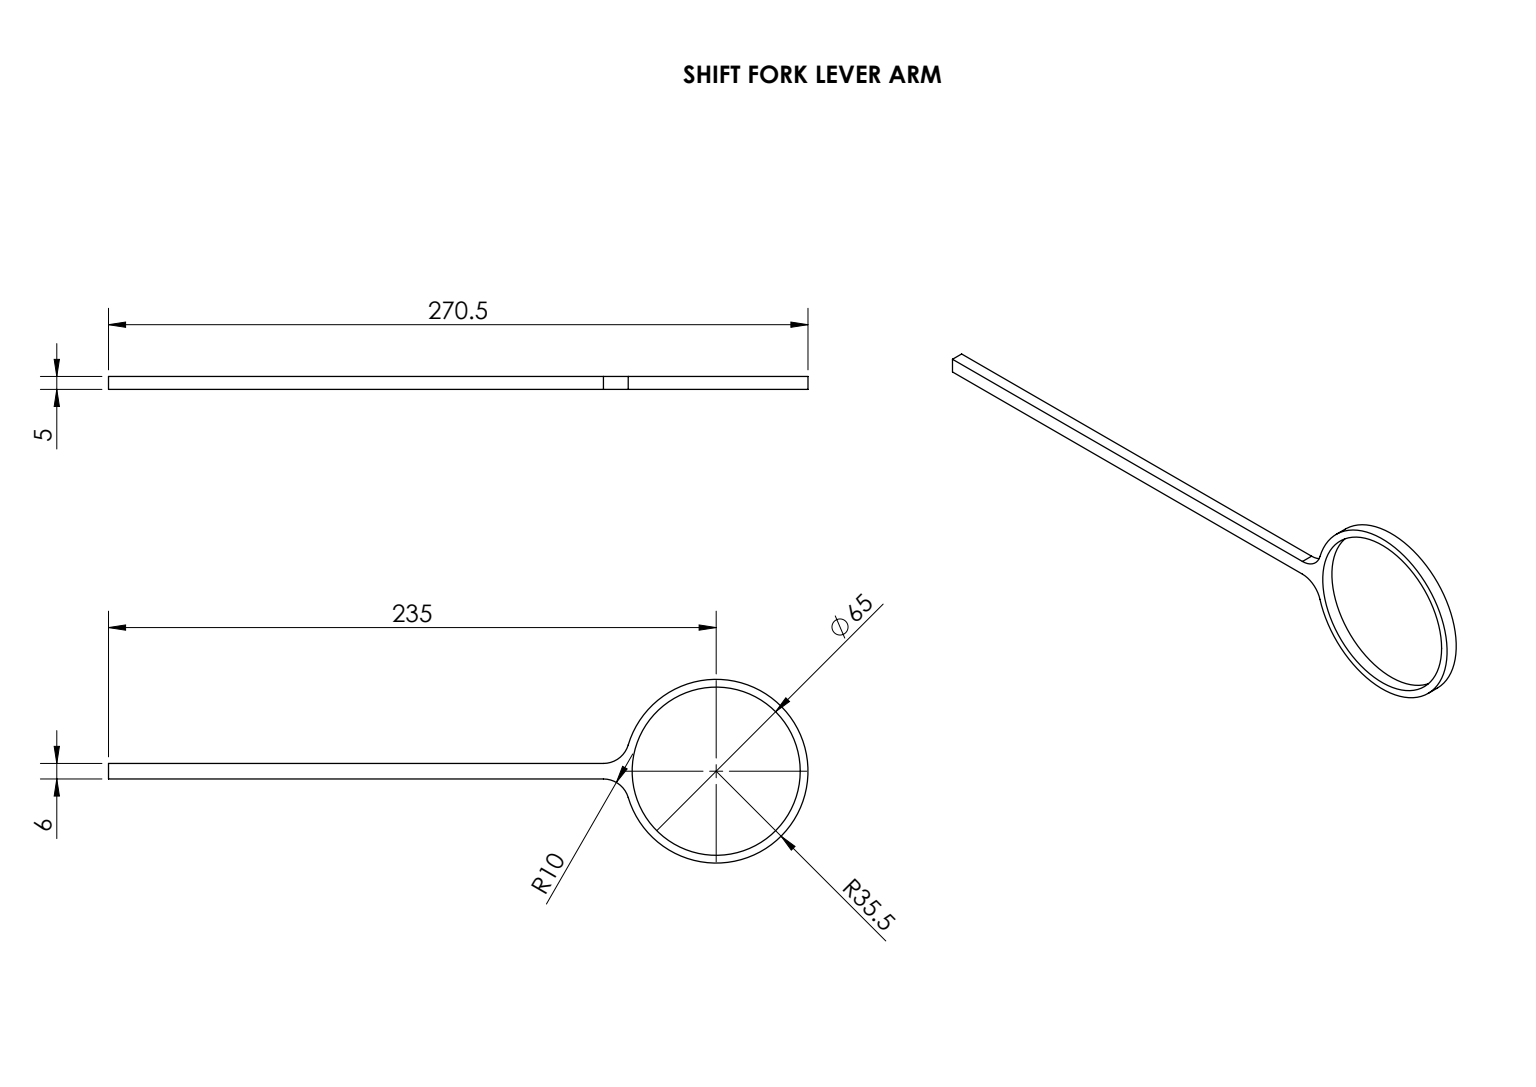
ISO-10303-21;
HEADER;
FILE_DESCRIPTION (('STEP AP214'),
    '1' );
FILE_NAME ('Shift Fork Lever Arm.step',
    '2026-10-08T09:53:37',
    ( '' ),
    ( '' ),
    'SwSTEP 2.0',
    'SolidWorks 2026',
    '' );
FILE_SCHEMA (( 'AUTOMOTIVE_DESIGN' ));
ENDSEC;

DATA;
#279=MECHANICAL_DESIGN_GEOMETRIC_PRESENTATION_REPRESENTATION('',(#31450),#13423);
#493=EDGE_CURVE ( 'NONE', #50397, #40961, #31739, .T. ) ;
#506=EDGE_LOOP ( 'NONE', ( #47657, #21524 ) ) ;
#1089=ORIENTED_EDGE ( 'NONE', *, *, #58225, .F. ) ;
#1094=VERTEX_POINT ( 'NONE', #69858 ) ;
#1250=ORIENTED_EDGE ( 'NONE', *, *, #69986, .F. ) ;
#1371=CARTESIAN_POINT ( 'NONE',  ( 0.000000000000000000, -120.0000000000000000, 2.500000000000000000 ) ) ;
#1832=ORIENTED_EDGE ( 'NONE', *, *, #65900, .T. ) ;
#1851=CARTESIAN_POINT ( 'NONE',  ( -35.37301231164799731, -123.0000000000000142, 2.500000000000000000 ) ) ;
#2124=PRESENTATION_STYLE_ASSIGNMENT (( #17159 ) ) ;
#2378=DIRECTION ( 'NONE',  ( 0.000000000000000000, 0.000000000000000000, -1.000000000000000000 ) ) ;
#2416=( NAMED_UNIT ( * ) PLANE_ANGLE_UNIT ( ) SI_UNIT ( $, .RADIAN. ) );
#2539=CARTESIAN_POINT ( 'NONE',  ( -43.60332556124591008, -133.0000000000000000, 2.500000000000002220 ) ) ;
#2571=DIRECTION ( 'NONE',  ( 0.000000000000000000, 0.000000000000000000, 1.000000000000000000 ) ) ;
#2729=ORIENTED_EDGE ( 'NONE', *, *, #17511, .F. ) ;
#2903=DIRECTION ( 'NONE',  ( -0.000000000000000000, -0.000000000000000000, -1.000000000000000000 ) ) ;
#2976=CARTESIAN_POINT ( 'NONE',  ( -43.60332556124591008, -123.0000000000000142, 2.500000000000000000 ) ) ;
#3170=PRODUCT_DEFINITION_SHAPE ( 'NONE', 'NONE',  #3585 ) ;
#3188=FACE_OUTER_BOUND ( 'NONE', #56711, .T. ) ;
#3275=ORIENTED_EDGE ( 'NONE', *, *, #38816, .F. ) ;
#3585=PRODUCT_DEFINITION ( 'UNKNOWN', '', #40042, #37882 ) ;
#3925=CARTESIAN_POINT ( 'NONE',  ( 0.000000000000000000, -120.0000000000000000, -2.500000000000000000 ) ) ;
#4365=EDGE_CURVE ( 'NONE', #9063, #35752, #34989, .T. ) ;
#4378=ORIENTED_EDGE ( 'NONE', *, *, #60273, .T. ) ;
#4546=VERTEX_POINT ( 'NONE', #31183 ) ;
#5317=ORIENTED_EDGE ( 'NONE', *, *, #5543, .T. ) ;
#5519=CIRCLE ( 'NONE', #39091, 35.50000000000000711 ) ;
#5524=FILL_AREA_STYLE ('',( #57018 ) ) ;
#5543=EDGE_CURVE ( 'NONE', #40961, #24049, #31285, .T. ) ;
#5914=AXIS2_PLACEMENT_3D ( 'NONE', #72472, #61583, #21719 ) ;
#6313=ORIENTED_EDGE ( 'NONE', *, *, #61943, .F. ) ;
#6345=CYLINDRICAL_SURFACE ( 'NONE', #60879, 10.00000000000000178 ) ;
#6694=CARTESIAN_POINT ( 'NONE',  ( 0.000000000000000000, -120.0000000000000000, 2.500000000000000000 ) ) ;
#6741=AXIS2_PLACEMENT_3D ( 'NONE', #9368, #48121, #71037 ) ;
#6882=DIRECTION ( 'NONE',  ( -0.000000000000000000, -0.000000000000000000, -1.000000000000000000 ) ) ;
#6961=AXIS2_PLACEMENT_3D ( 'NONE', #15987, #28005, #39680 ) ;
#7060=EDGE_CURVE ( 'NONE', #1094, #43028, #54701, .T. ) ;
#7091=DIRECTION ( 'NONE',  ( -0.000000000000000000, -0.000000000000000000, -1.000000000000000000 ) ) ;
#7468=EDGE_CURVE ( 'NONE', #56318, #9063, #47331, .T. ) ;
#7900=DIRECTION ( 'NONE',  ( -0.000000000000000000, -0.000000000000000000, -1.000000000000000000 ) ) ;
#7939=ORIENTED_EDGE ( 'NONE', *, *, #55262, .F. ) ;
#7967=CARTESIAN_POINT ( 'NONE',  ( -235.0000123116479926, -123.0000000000000284, 2.500000000000000000 ) ) ;
#8007=SHAPE_REPRESENTATION_RELATIONSHIP ( 'NONE' , 'NONE' ,  #54059, #64162 ) ;
#8296=AXIS2_PLACEMENT_3D ( 'NONE', #54037, #2571, #25454 ) ;
#8331=ORIENTED_EDGE ( 'NONE', *, *, #55262, .T. ) ;
#8584=ORIENTED_EDGE ( 'NONE', *, *, #493, .F. ) ;
#8605=ORIENTED_EDGE ( 'NONE', *, *, #53404, .F. ) ;
#8753=( NAMED_UNIT ( * ) SI_UNIT ( $, .STERADIAN. ) SOLID_ANGLE_UNIT ( ) );
#9036=DIRECTION ( 'NONE',  ( -1.000000000000000000, -1.390371824233641368E-16, 0.000000000000000000 ) ) ;
#9063=VERTEX_POINT ( 'NONE', #38613 ) ;
#9368=CARTESIAN_POINT ( 'NONE',  ( 0.000000000000000000, -89.50000000000000000, 2.500000000000000000 ) ) ;
#9389=AXIS2_PLACEMENT_3D ( 'NONE', #63819, #22857, #29567 ) ;
#9403=CARTESIAN_POINT ( 'NONE',  ( -35.37301231164799731, -117.0000000000000000, 2.500000000000000000 ) ) ;
#9425=AXIS2_PLACEMENT_3D ( 'NONE', #65440, #18807, #41748 ) ;
#9496=AXIS2_PLACEMENT_3D ( 'NONE', #7967, #30884, #2378 ) ;
#9669=CARTESIAN_POINT ( 'NONE',  ( -43.60332556124591719, -107.0000000000000000, -2.500000000000002220 ) ) ;
#10522=STYLED_ITEM ( 'NONE', ( #2124 ), #12416 ) ;
#11005=PRODUCT ( 'Shift Fork Lever Arm', 'Shift Fork Lever Arm', '', ( #62921 ) ) ;
#11567=DIRECTION ( 'NONE',  ( 1.000000000000000000, 0.000000000000000000, 0.000000000000000000 ) ) ;
#11920=FACE_OUTER_BOUND ( 'NONE', #33954, .T. ) ;
#12163=( NAMED_UNIT ( * ) PLANE_ANGLE_UNIT ( ) SI_UNIT ( $, .RADIAN. ) );
#12416=MANIFOLD_SOLID_BREP ( 'Fillet1', #39184 ) ;
#12418=DIRECTION ( 'NONE',  ( -0.000000000000000000, -0.000000000000000000, -1.000000000000000000 ) ) ;
#12755=CARTESIAN_POINT ( 'NONE',  ( -34.02017708624681092, -109.8571428571428470, -2.500000000000000000 ) ) ;
#12885=VECTOR ( 'NONE', #6882, 1000.000000000000000 ) ;
#12983=DIRECTION ( 'NONE',  ( 0.000000000000000000, 0.000000000000000000, -1.000000000000000000 ) ) ;
#13364=CARTESIAN_POINT ( 'NONE',  ( -43.60332556124591719, -107.0000000000000000, 2.500000000000002220 ) ) ;
#13423=( GEOMETRIC_REPRESENTATION_CONTEXT ( 3 ) GLOBAL_UNCERTAINTY_ASSIGNED_CONTEXT ( ( #50455 ) ) GLOBAL_UNIT_ASSIGNED_CONTEXT ( ( #48956, #2416, #59522 ) ) REPRESENTATION_CONTEXT ( 'NONE', 'WORKASPACE' ) );
#13429=FACE_OUTER_BOUND ( 'NONE', #53169, .T. ) ;
#13605=PLANE ( 'NONE',  #9496 ) ;
#13638=PRESENTATION_STYLE_ASSIGNMENT (( #53869 ) ) ;
#13734=CARTESIAN_POINT ( 'NONE',  ( 32.50000000000000000, -120.0000000000000000, -2.500000000000000000 ) ) ;
#13827=FACE_OUTER_BOUND ( 'NONE', #32175, .T. ) ;
#14831=ORIENTED_EDGE ( 'NONE', *, *, #7468, .F. ) ;
#15138=CARTESIAN_POINT ( 'NONE',  ( -235.0000123116479926, -117.0000000000000142, -2.500000000000000000 ) ) ;
#15313=ORIENTED_EDGE ( 'NONE', *, *, #60273, .F. ) ;
#15737=DIRECTION ( 'NONE',  ( 0.000000000000000000, 0.000000000000000000, 1.000000000000000000 ) ) ;
#15987=CARTESIAN_POINT ( 'NONE',  ( 0.000000000000000000, -120.0000000000000000, -2.500000000000000000 ) ) ;
#16227=CARTESIAN_POINT ( 'NONE',  ( -43.60332556124591008, -133.0000000000000000, -2.500000000000002220 ) ) ;
#16229=VECTOR ( 'NONE', #7091, 1000.000000000000000 ) ;
#16483=ORIENTED_EDGE ( 'NONE', *, *, #53404, .T. ) ;
#16593=VECTOR ( 'NONE', #2903, 1000.000000000000000 ) ;
#17053=DIRECTION ( 'NONE',  ( 0.000000000000000000, 0.000000000000000000, 1.000000000000000000 ) ) ;
#17123=ORIENTED_EDGE ( 'NONE', *, *, #45687, .T. ) ;
#17159=SURFACE_STYLE_USAGE ( .BOTH. , #45751 ) ;
#17215=ORIENTED_EDGE ( 'NONE', *, *, #73567, .F. ) ;
#17511=EDGE_CURVE ( 'NONE', #56318, #50947, #63362, .T. ) ;
#17619=DIRECTION ( 'NONE',  ( 1.000000000000000000, 0.000000000000000000, 0.000000000000000000 ) ) ;
#17699=CIRCLE ( 'NONE', #29699, 10.00000000000000178 ) ;
#18203=VECTOR ( 'NONE', #7900, 1000.000000000000000 ) ;
#18807=DIRECTION ( 'NONE',  ( -0.000000000000000000, -0.000000000000000000, -1.000000000000000000 ) ) ;
#19275=AXIS2_PLACEMENT_3D ( 'NONE', #57478, #33799, #17619 ) ;
#19553=CYLINDRICAL_SURFACE ( 'NONE', #9425, 35.50000000000001421 ) ;
#19735=DIRECTION ( 'NONE',  ( 1.000000000000000000, 0.000000000000000000, 0.000000000000000000 ) ) ;
#19776=LINE ( 'NONE', #25796, #16593 ) ;
#20065=PLANE ( 'NONE',  #27557 ) ;
#20255=EDGE_LOOP ( 'NONE', ( #14831, #49366 ) ) ;
#20263=EDGE_CURVE ( 'NONE', #9063, #56318, #59292, .T. ) ;
#20939=CARTESIAN_POINT ( 'NONE',  ( -32.50000000000000000, -120.0000000000000000, 2.500000000000000000 ) ) ;
#21420=VERTEX_POINT ( 'NONE', #32289 ) ;
#21524=ORIENTED_EDGE ( 'NONE', *, *, #39635, .T. ) ;
#21649=EDGE_LOOP ( 'NONE', ( #30424, #45563, #40231, #31968 ) ) ;
#21719=DIRECTION ( 'NONE',  ( -1.000000000000000000, 0.000000000000000000, 0.000000000000000000 ) ) ;
#21767=VECTOR ( 'NONE', #17053, 1000.000000000000000 ) ;
#21935=ORIENTED_EDGE ( 'NONE', *, *, #38816, .T. ) ;
#22048=CARTESIAN_POINT ( 'NONE',  ( -235.0000123116479926, -123.0000000000000284, 2.500000000000000000 ) ) ;
#22559=AXIS2_PLACEMENT_3D ( 'NONE', #13364, #12983, #35192 ) ;
#22594=EDGE_CURVE ( 'NONE', #4546, #21420, #31199, .T. ) ;
#22857=DIRECTION ( 'NONE',  ( -0.000000000000000000, -0.000000000000000000, -1.000000000000000000 ) ) ;
#23041=EDGE_CURVE ( 'NONE', #43028, #24049, #30369, .T. ) ;
#23084=EDGE_CURVE ( 'NONE', #21420, #53605, #42404, .T. ) ;
#23107=VECTOR ( 'NONE', #47667, 1000.000000000000000 ) ;
#23205=LINE ( 'NONE', #46135, #54644 ) ;
#23986=ORIENTED_EDGE ( 'NONE', *, *, #29706, .T. ) ;
#24049=VERTEX_POINT ( 'NONE', #2976 ) ;
#24262=DIRECTION ( 'NONE',  ( -0.000000000000000000, -0.000000000000000000, 1.000000000000000000 ) ) ;
#24645=CARTESIAN_POINT ( 'NONE',  ( -34.02017708624681092, -130.1428571428571388, -2.500000000000000000 ) ) ;
#24747=LINE ( 'NONE', #53692, #16229 ) ;
#25045=DIRECTION ( 'NONE',  ( 0.000000000000000000, 0.000000000000000000, -1.000000000000000000 ) ) ;
#25193=FACE_OUTER_BOUND ( 'NONE', #47030, .T. ) ;
#25355=CARTESIAN_POINT ( 'NONE',  ( -35.37301231164799731, -123.0000000000000142, 2.500000000000000000 ) ) ;
#25454=DIRECTION ( 'NONE',  ( 1.000000000000000000, 0.000000000000000000, -0.000000000000000000 ) ) ;
#25796=CARTESIAN_POINT ( 'NONE',  ( -34.02017708624681092, -130.1428571428571388, 102.9091629284897493 ) ) ;
#26391=CARTESIAN_POINT ( 'NONE',  ( -43.60332556124591008, -123.0000000000000142, 2.500000000000002220 ) ) ;
#26624=ADVANCED_FACE ( 'NONE', ( #46958 ), #57871, .F. ) ;
#26658=PLANE ( 'NONE',  #6741 ) ;
#27539=VERTEX_POINT ( 'NONE', #42849 ) ;
#27557=AXIS2_PLACEMENT_3D ( 'NONE', #25355, #49009, #59951 ) ;
#28005=DIRECTION ( 'NONE',  ( 0.000000000000000000, 0.000000000000000000, 1.000000000000000000 ) ) ;
#29242=CARTESIAN_POINT ( 'NONE',  ( -43.60332556124591719, -107.0000000000000000, 102.9091629284897493 ) ) ;
#29424=EDGE_CURVE ( 'NONE', #21420, #54327, #63412, .T. ) ;
#29567=DIRECTION ( 'NONE',  ( -1.000000000000000000, 0.000000000000000000, 0.000000000000000000 ) ) ;
#29699=AXIS2_PLACEMENT_3D ( 'NONE', #2539, #25045, #70898 ) ;
#29706=EDGE_CURVE ( 'NONE', #59857, #4546, #36986, .T. ) ;
#29946=ORIENTED_EDGE ( 'NONE', *, *, #7060, .T. ) ;
#29999=CARTESIAN_POINT ( 'NONE',  ( -35.37301231164799731, -117.0000000000000000, -2.500000000000000000 ) ) ;
#30369=LINE ( 'NONE', #1851, #31498 ) ;
#30424=ORIENTED_EDGE ( 'NONE', *, *, #4365, .F. ) ;
#30637=( NAMED_UNIT ( * ) PLANE_ANGLE_UNIT ( ) SI_UNIT ( $, .RADIAN. ) );
#30884=DIRECTION ( 'NONE',  ( 1.000000000000000000, 0.000000000000000000, 0.000000000000000000 ) ) ;
#31082=PLANE ( 'NONE',  #8296 ) ;
#31183=CARTESIAN_POINT ( 'NONE',  ( -43.60332556124591719, -117.0000000000000000, 2.500000000000000000 ) ) ;
#31199=LINE ( 'NONE', #65434, #18203 ) ;
#31285=LINE ( 'NONE', #26391, #73974 ) ;
#31321=ORIENTED_EDGE ( 'NONE', *, *, #23041, .F. ) ;
#31450=STYLED_ITEM ( 'NONE', ( #13638 ), #64162 ) ;
#31483=DIRECTION ( 'NONE',  ( 1.000000000000000000, 0.000000000000000000, 0.000000000000000000 ) ) ;
#31498=VECTOR ( 'NONE', #70576, 1000.000000000000000 ) ;
#31739=CIRCLE ( 'NONE', #68847, 10.00000000000000178 ) ;
#31943=AXIS2_PLACEMENT_3D ( 'NONE', #36032, #69871, #34554 ) ;
#31968=ORIENTED_EDGE ( 'NONE', *, *, #39635, .F. ) ;
#32031=CARTESIAN_POINT ( 'NONE',  ( -32.50000000000000000, -120.0000000000000000, -2.500000000000000000 ) ) ;
#32104=ORIENTED_EDGE ( 'NONE', *, *, #61943, .T. ) ;
#32175=EDGE_LOOP ( 'NONE', ( #3275, #64817, #8584, #73597 ) ) ;
#32271=VECTOR ( 'NONE', #9036, 1000.000000000000000 ) ;
#32289=CARTESIAN_POINT ( 'NONE',  ( -43.60332556124591719, -117.0000000000000000, -2.500000000000000000 ) ) ;
#32953=DIRECTION ( 'NONE',  ( 0.000000000000000000, 0.000000000000000000, 1.000000000000000000 ) ) ;
#33592=ADVANCED_FACE ( 'NONE', ( #73214 ), #66484, .F. ) ;
#33799=DIRECTION ( 'NONE',  ( 0.000000000000000000, 0.000000000000000000, 1.000000000000000000 ) ) ;
#33954=EDGE_LOOP ( 'NONE', ( #63918, #44488, #17215, #2729 ) ) ;
#33966=LINE ( 'NONE', #34335, #21767 ) ;
#34335=CARTESIAN_POINT ( 'NONE',  ( -34.02017708624681092, -109.8571428571428470, 102.9091629284897493 ) ) ;
#34554=DIRECTION ( 'NONE',  ( 1.000000000000000000, 1.390371824233641368E-16, 0.000000000000000000 ) ) ;
#34574=UNCERTAINTY_MEASURE_WITH_UNIT (LENGTH_MEASURE( 1.000000000000000082E-05 ), #70864, 'distance_accuracy_value', 'NONE');
#34601=ORIENTED_EDGE ( 'NONE', *, *, #22594, .F. ) ;
#34780=CARTESIAN_POINT ( 'NONE',  ( -32.50000000000000000, -120.0000000000000000, 102.9091629284897493 ) ) ;
#34904=DIRECTION ( 'NONE',  ( -1.000000000000000000, 0.000000000000000000, 0.000000000000000000 ) ) ;
#34989=LINE ( 'NONE', #51532, #54228 ) ;
#35192=DIRECTION ( 'NONE',  ( 1.000000000000000000, 1.387778780781445478E-15, 0.000000000000000000 ) ) ;
#35497=ORIENTED_EDGE ( 'NONE', *, *, #69986, .T. ) ;
#35620=DIRECTION ( 'NONE',  ( 0.000000000000000000, 0.000000000000000000, 1.000000000000000000 ) ) ;
#35752=VERTEX_POINT ( 'NONE', #13734 ) ;
#36032=CARTESIAN_POINT ( 'NONE',  ( -35.37301231164799731, -117.0000000000000000, 2.500000000000000000 ) ) ;
#36052=ORIENTED_EDGE ( 'NONE', *, *, #22594, .T. ) ;
#36427=APPLICATION_CONTEXT ( 'automotive_design' ) ;
#36986=CIRCLE ( 'NONE', #22559, 10.00000000000000178 ) ;
#37527=DIRECTION ( 'NONE',  ( -1.000000000000000000, 0.000000000000000000, 0.000000000000000000 ) ) ;
#37587=FACE_BOUND ( 'NONE', #20255, .T. ) ;
#37882=PRODUCT_DEFINITION_CONTEXT ( 'detailed design', #44125, 'design' ) ;
#38097=ORIENTED_EDGE ( 'NONE', *, *, #23041, .T. ) ;
#38460=ORIENTED_EDGE ( 'NONE', *, *, #23084, .F. ) ;
#38613=CARTESIAN_POINT ( 'NONE',  ( 32.50000000000000000, -120.0000000000000000, 2.500000000000000000 ) ) ;
#38730=LINE ( 'NONE', #9403, #32271 ) ;
#38816=EDGE_CURVE ( 'NONE', #24049, #27539, #17699, .T. ) ;
#39091=AXIS2_PLACEMENT_3D ( 'NONE', #1371, #24262, #53942 ) ;
#39184=CLOSED_SHELL ( 'NONE', ( #62589, #43492, #40828, #33592, #66730, #26624, #64979, #46346, #71158, #61555 ) ) ;
#39364=MECHANICAL_DESIGN_GEOMETRIC_PRESENTATION_REPRESENTATION('',(#10522),#68180);
#39635=EDGE_CURVE ( 'NONE', #35752, #50947, #72939, .T. ) ;
#39680=DIRECTION ( 'NONE',  ( 1.000000000000000000, 0.000000000000000000, 0.000000000000000000 ) ) ;
#40027=ORIENTED_EDGE ( 'NONE', *, *, #29706, .F. ) ;
#40042=PRODUCT_DEFINITION_FORMATION_WITH_SPECIFIED_SOURCE ( 'ANY', '', #11005, .NOT_KNOWN. ) ;
#40231=ORIENTED_EDGE ( 'NONE', *, *, #17511, .T. ) ;
#40482=DIRECTION ( 'NONE',  ( -0.000000000000000000, -1.000000000000000000, -0.000000000000000000 ) ) ;
#40537=FACE_OUTER_BOUND ( 'NONE', #50098, .T. ) ;
#40828=ADVANCED_FACE ( 'NONE', ( #13429, #59672 ), #31082, .F. ) ;
#40961=VERTEX_POINT ( 'NONE', #72419 ) ;
#41077=SHAPE_DEFINITION_REPRESENTATION ( #3170, #54059 ) ;
#41165=DIRECTION ( 'NONE',  ( -0.000000000000000000, -0.000000000000000000, -1.000000000000000000 ) ) ;
#41265=AXIS2_PLACEMENT_3D ( 'NONE', #73609, #15737, #11567 ) ;
#41748=DIRECTION ( 'NONE',  ( -1.000000000000000000, 0.000000000000000000, 0.000000000000000000 ) ) ;
#42404=LINE ( 'NONE', #29999, #23107 ) ;
#42849=CARTESIAN_POINT ( 'NONE',  ( -34.02017708624680381, -130.1428571428571388, 2.500000000000000000 ) ) ;
#42964=COLOUR_RGB ( '', 0.40784314, 0.44705882, 0.49803922) ;
#43028=VERTEX_POINT ( 'NONE', #47129 ) ;
#43395=AXIS2_PLACEMENT_3D ( 'NONE', #48320, #71232, #19735 ) ;
#43492=ADVANCED_FACE ( 'NONE', ( #71049 ), #19553, .T. ) ;
#44125=APPLICATION_CONTEXT ( 'automotive_design' ) ;
#44461=UNCERTAINTY_MEASURE_WITH_UNIT (LENGTH_MEASURE( 1.000000000000000082E-05 ), #46761, 'distance_accuracy_value', 'NONE');
#44488=ORIENTED_EDGE ( 'NONE', *, *, #4365, .T. ) ;
#45563=ORIENTED_EDGE ( 'NONE', *, *, #20263, .T. ) ;
#45687=EDGE_CURVE ( 'NONE', #4546, #1094, #38730, .T. ) ;
#45751=SURFACE_SIDE_STYLE ('',( #74298 ) ) ;
#45865=( GEOMETRIC_REPRESENTATION_CONTEXT ( 3 ) GLOBAL_UNCERTAINTY_ASSIGNED_CONTEXT ( ( #44461 ) ) GLOBAL_UNIT_ASSIGNED_CONTEXT ( ( #46761, #12163, #8753 ) ) REPRESENTATION_CONTEXT ( 'NONE', 'WORKASPACE' ) );
#45963=ORIENTED_EDGE ( 'NONE', *, *, #493, .T. ) ;
#46135=CARTESIAN_POINT ( 'NONE',  ( -235.0000123116479926, -123.0000000000000284, -2.500000000000000000 ) ) ;
#46346=ADVANCED_FACE ( 'NONE', ( #3188 ), #20065, .F. ) ;
#46511=CYLINDRICAL_SURFACE ( 'NONE', #9389, 32.50000000000000000 ) ;
#46761=( LENGTH_UNIT ( ) NAMED_UNIT ( * ) SI_UNIT ( .MILLI., .METRE. ) );
#46835=VERTEX_POINT ( 'NONE', #54573 ) ;
#46958=FACE_OUTER_BOUND ( 'NONE', #58505, .T. ) ;
#47030=EDGE_LOOP ( 'NONE', ( #38097, #21935, #4378, #23986, #17123, #29946 ) ) ;
#47129=CARTESIAN_POINT ( 'NONE',  ( -235.0000123116479926, -123.0000000000000284, 2.500000000000000000 ) ) ;
#47331=CIRCLE ( 'NONE', #60547, 32.50000000000000000 ) ;
#47657=ORIENTED_EDGE ( 'NONE', *, *, #73567, .T. ) ;
#47667=DIRECTION ( 'NONE',  ( -1.000000000000000000, -1.390371824233641368E-16, 0.000000000000000000 ) ) ;
#48121=DIRECTION ( 'NONE',  ( 0.000000000000000000, -0.000000000000000000, 1.000000000000000000 ) ) ;
#48236=SURFACE_STYLE_FILL_AREA ( #60634 ) ;
#48320=CARTESIAN_POINT ( 'NONE',  ( 0.000000000000000000, 0.000000000000000000, 0.000000000000000000 ) ) ;
#48603=FILL_AREA_STYLE_COLOUR ( '', #61470 ) ;
#48956=( LENGTH_UNIT ( ) NAMED_UNIT ( * ) SI_UNIT ( .MILLI., .METRE. ) );
#49009=DIRECTION ( 'NONE',  ( -6.951859121168206841E-17, 1.000000000000000000, 0.000000000000000000 ) ) ;
#49112=CARTESIAN_POINT ( 'NONE',  ( -34.02017708624680381, -109.8571428571428470, 2.500000000000000000 ) ) ;
#49164=DIRECTION ( 'NONE',  ( -0.000000000000000000, -0.000000000000000000, -1.000000000000000000 ) ) ;
#49366=ORIENTED_EDGE ( 'NONE', *, *, #20263, .F. ) ;
#50098=EDGE_LOOP ( 'NONE', ( #40027, #51577, #62462, #34601 ) ) ;
#50397=VERTEX_POINT ( 'NONE', #24645 ) ;
#50455=UNCERTAINTY_MEASURE_WITH_UNIT (LENGTH_MEASURE( 1.000000000000000082E-05 ), #48956, 'distance_accuracy_value', 'NONE');
#50947=VERTEX_POINT ( 'NONE', #32031 ) ;
#51143=ORIENTED_EDGE ( 'NONE', *, *, #29424, .T. ) ;
#51532=CARTESIAN_POINT ( 'NONE',  ( 32.50000000000000000, -120.0000000000000000, 102.9091629284897493 ) ) ;
#51577=ORIENTED_EDGE ( 'NONE', *, *, #65900, .F. ) ;
#51861=VECTOR ( 'NONE', #41165, 1000.000000000000000 ) ;
#52291=DIRECTION ( 'NONE',  ( 0.000000000000000000, 0.000000000000000000, 1.000000000000000000 ) ) ;
#52323=ORIENTED_EDGE ( 'NONE', *, *, #45687, .F. ) ;
#52465=( NAMED_UNIT ( * ) SI_UNIT ( $, .STERADIAN. ) SOLID_ANGLE_UNIT ( ) );
#53169=EDGE_LOOP ( 'NONE', ( #7939, #45963, #1250, #8605, #38460, #51143 ) ) ;
#53404=EDGE_CURVE ( 'NONE', #53605, #46835, #23205, .T. ) ;
#53488=DIRECTION ( 'NONE',  ( 0.000000000000000000, 0.000000000000000000, 1.000000000000000000 ) ) ;
#53605=VERTEX_POINT ( 'NONE', #15138 ) ;
#53692=CARTESIAN_POINT ( 'NONE',  ( -235.0000123116479926, -117.0000000000000142, 2.500000000000000000 ) ) ;
#53869=SURFACE_STYLE_USAGE ( .BOTH. , #72260 ) ;
#53934=DIRECTION ( 'NONE',  ( 1.000000000000000000, 0.000000000000000000, 0.000000000000000000 ) ) ;
#53942=DIRECTION ( 'NONE',  ( 1.000000000000000000, 0.000000000000000000, 0.000000000000000000 ) ) ;
#54037=CARTESIAN_POINT ( 'NONE',  ( 0.000000000000000000, -120.0000000000000000, -2.500000000000000000 ) ) ;
#54059=SHAPE_REPRESENTATION ( 'Shift Fork Lever Arm', ( #43395 ), #45865 ) ;
#54228=VECTOR ( 'NONE', #12418, 1000.000000000000000 ) ;
#54327=VERTEX_POINT ( 'NONE', #12755 ) ;
#54573=CARTESIAN_POINT ( 'NONE',  ( -235.0000123116479926, -123.0000000000000284, -2.500000000000000000 ) ) ;
#54644=VECTOR ( 'NONE', #40482, 1000.000000000000000 ) ;
#54701=LINE ( 'NONE', #67087, #64090 ) ;
#55136=AXIS2_PLACEMENT_3D ( 'NONE', #66467, #49164, #37527 ) ;
#55209=ORIENTED_EDGE ( 'NONE', *, *, #62701, .T. ) ;
#55262=EDGE_CURVE ( 'NONE', #50397, #54327, #72310, .T. ) ;
#55281=CIRCLE ( 'NONE', #19275, 32.50000000000000000 ) ;
#55540=DIRECTION ( 'NONE',  ( 1.000000000000000000, 6.951859121168206841E-17, -0.000000000000000000 ) ) ;
#56207=AXIS2_PLACEMENT_3D ( 'NONE', #9669, #32953, #31483 ) ;
#56318=VERTEX_POINT ( 'NONE', #20939 ) ;
#56711=EDGE_LOOP ( 'NONE', ( #35497, #5317, #31321, #32104 ) ) ;
#57018=FILL_AREA_STYLE_COLOUR ( '', #42964 ) ;
#57153=ORIENTED_EDGE ( 'NONE', *, *, #7060, .F. ) ;
#57478=CARTESIAN_POINT ( 'NONE',  ( 0.000000000000000000, -120.0000000000000000, -2.500000000000000000 ) ) ;
#57871=PLANE ( 'NONE',  #31943 ) ;
#58225=EDGE_CURVE ( 'NONE', #1094, #53605, #24747, .T. ) ;
#58505=EDGE_LOOP ( 'NONE', ( #52323, #36052, #61309, #1089 ) ) ;
#58768=LINE ( 'NONE', #22048, #12885 ) ;
#58832=EDGE_LOOP ( 'NONE', ( #15313, #55209, #8331, #1832 ) ) ;
#59071=AXIS2_PLACEMENT_3D ( 'NONE', #3925, #61046, #53934 ) ;
#59292=CIRCLE ( 'NONE', #41265, 32.50000000000000000 ) ;
#59522=( NAMED_UNIT ( * ) SI_UNIT ( $, .STERADIAN. ) SOLID_ANGLE_UNIT ( ) );
#59672=FACE_BOUND ( 'NONE', #506, .T. ) ;
#59799=CARTESIAN_POINT ( 'NONE',  ( -35.37301231164799731, -123.0000000000000142, -2.500000000000000000 ) ) ;
#59857=VERTEX_POINT ( 'NONE', #49112 ) ;
#59951=DIRECTION ( 'NONE',  ( -1.000000000000000000, -6.951859121168206841E-17, 0.000000000000000000 ) ) ;
#60273=EDGE_CURVE ( 'NONE', #27539, #59857, #5519, .T. ) ;
#60547=AXIS2_PLACEMENT_3D ( 'NONE', #6694, #35620, #70194 ) ;
#60634=FILL_AREA_STYLE ('',( #48603 ) ) ;
#60879=AXIS2_PLACEMENT_3D ( 'NONE', #29242, #62383, #34904 ) ;
#61046=DIRECTION ( 'NONE',  ( 0.000000000000000000, 0.000000000000000000, 1.000000000000000000 ) ) ;
#61309=ORIENTED_EDGE ( 'NONE', *, *, #23084, .T. ) ;
#61470=COLOUR_RGB ( '', 0.40784314, 0.44705882, 0.49803922) ;
#61555=ADVANCED_FACE ( 'NONE', ( #40537 ), #6345, .F. ) ;
#61583=DIRECTION ( 'NONE',  ( -0.000000000000000000, -0.000000000000000000, -1.000000000000000000 ) ) ;
#61943=EDGE_CURVE ( 'NONE', #43028, #46835, #58768, .T. ) ;
#62230=VECTOR ( 'NONE', #55540, 1000.000000000000000 ) ;
#62383=DIRECTION ( 'NONE',  ( -0.000000000000000000, -0.000000000000000000, -1.000000000000000000 ) ) ;
#62462=ORIENTED_EDGE ( 'NONE', *, *, #29424, .F. ) ;
#62589=ADVANCED_FACE ( 'NONE', ( #11920 ), #46511, .F. ) ;
#62701=EDGE_CURVE ( 'NONE', #27539, #50397, #19776, .T. ) ;
#62921=PRODUCT_CONTEXT ( 'NONE', #36427, 'mechanical' ) ;
#63223=DIRECTION ( 'NONE',  ( 1.000000000000000000, 0.000000000000000000, 0.000000000000000000 ) ) ;
#63362=LINE ( 'NONE', #34780, #51861 ) ;
#63412=CIRCLE ( 'NONE', #56207, 10.00000000000000178 ) ;
#63819=CARTESIAN_POINT ( 'NONE',  ( 0.000000000000000000, -120.0000000000000000, 102.9091629284897493 ) ) ;
#63918=ORIENTED_EDGE ( 'NONE', *, *, #7468, .T. ) ;
#64090=VECTOR ( 'NONE', #72706, 1000.000000000000000 ) ;
#64162=ADVANCED_BREP_SHAPE_REPRESENTATION ( '', ( #12416, #43395 ), #45865 ) ;
#64817=ORIENTED_EDGE ( 'NONE', *, *, #5543, .F. ) ;
#64901=ORIENTED_EDGE ( 'NONE', *, *, #58225, .T. ) ;
#64979=ADVANCED_FACE ( 'NONE', ( #65128 ), #13605, .F. ) ;
#65128=FACE_OUTER_BOUND ( 'NONE', #67896, .T. ) ;
#65434=CARTESIAN_POINT ( 'NONE',  ( -43.60332556124591719, -117.0000000000000000, -2.500000000000002220 ) ) ;
#65440=CARTESIAN_POINT ( 'NONE',  ( 0.000000000000000000, -120.0000000000000000, 102.9091629284897493 ) ) ;
#65900=EDGE_CURVE ( 'NONE', #54327, #59857, #33966, .T. ) ;
#66467=CARTESIAN_POINT ( 'NONE',  ( -43.60332556124591008, -133.0000000000000000, 102.9091629284897493 ) ) ;
#66484=CYLINDRICAL_SURFACE ( 'NONE', #5914, 32.50000000000000000 ) ;
#66730=ADVANCED_FACE ( 'NONE', ( #37587, #25193 ), #26658, .T. ) ;
#67087=CARTESIAN_POINT ( 'NONE',  ( -235.0000123116479926, -123.0000000000000284, 2.500000000000000000 ) ) ;
#67896=EDGE_LOOP ( 'NONE', ( #16483, #6313, #57153, #64901 ) ) ;
#68180=( GEOMETRIC_REPRESENTATION_CONTEXT ( 3 ) GLOBAL_UNCERTAINTY_ASSIGNED_CONTEXT ( ( #34574 ) ) GLOBAL_UNIT_ASSIGNED_CONTEXT ( ( #70864, #30637, #52465 ) ) REPRESENTATION_CONTEXT ( 'NONE', 'WORKASPACE' ) );
#68847=AXIS2_PLACEMENT_3D ( 'NONE', #16227, #52291, #63223 ) ;
#69858=CARTESIAN_POINT ( 'NONE',  ( -235.0000123116479926, -117.0000000000000142, 2.500000000000000000 ) ) ;
#69871=DIRECTION ( 'NONE',  ( 1.390371824233641368E-16, -1.000000000000000000, 0.000000000000000000 ) ) ;
#69986=EDGE_CURVE ( 'NONE', #46835, #40961, #71418, .T. ) ;
#70194=DIRECTION ( 'NONE',  ( 1.000000000000000000, 0.000000000000000000, 0.000000000000000000 ) ) ;
#70576=DIRECTION ( 'NONE',  ( 1.000000000000000000, 6.951859121168206841E-17, -0.000000000000000000 ) ) ;
#70864=( LENGTH_UNIT ( ) NAMED_UNIT ( * ) SI_UNIT ( .MILLI., .METRE. ) );
#70898=DIRECTION ( 'NONE',  ( 1.000000000000000000, 0.000000000000000000, 0.000000000000000000 ) ) ;
#71037=DIRECTION ( 'NONE',  ( 1.000000000000000000, 0.000000000000000000, 0.000000000000000000 ) ) ;
#71049=FACE_OUTER_BOUND ( 'NONE', #58832, .T. ) ;
#71158=ADVANCED_FACE ( 'NONE', ( #13827 ), #71711, .F. ) ;
#71232=DIRECTION ( 'NONE',  ( 0.000000000000000000, 0.000000000000000000, 1.000000000000000000 ) ) ;
#71418=LINE ( 'NONE', #59799, #62230 ) ;
#71711=CYLINDRICAL_SURFACE ( 'NONE', #55136, 10.00000000000000178 ) ;
#72260=SURFACE_SIDE_STYLE ('',( #48236 ) ) ;
#72310=CIRCLE ( 'NONE', #59071, 35.50000000000001421 ) ;
#72419=CARTESIAN_POINT ( 'NONE',  ( -43.60332556124591008, -123.0000000000000142, -2.500000000000000000 ) ) ;
#72472=CARTESIAN_POINT ( 'NONE',  ( 0.000000000000000000, -120.0000000000000000, 102.9091629284897493 ) ) ;
#72706=DIRECTION ( 'NONE',  ( -0.000000000000000000, -1.000000000000000000, -0.000000000000000000 ) ) ;
#72939=CIRCLE ( 'NONE', #6961, 32.50000000000000000 ) ;
#73214=FACE_OUTER_BOUND ( 'NONE', #21649, .T. ) ;
#73567=EDGE_CURVE ( 'NONE', #50947, #35752, #55281, .T. ) ;
#73597=ORIENTED_EDGE ( 'NONE', *, *, #62701, .F. ) ;
#73609=CARTESIAN_POINT ( 'NONE',  ( 0.000000000000000000, -120.0000000000000000, 2.500000000000000000 ) ) ;
#73974=VECTOR ( 'NONE', #53488, 1000.000000000000000 ) ;
#74298=SURFACE_STYLE_FILL_AREA ( #5524 ) ;
ENDSEC;
END-ISO-10303-21;
